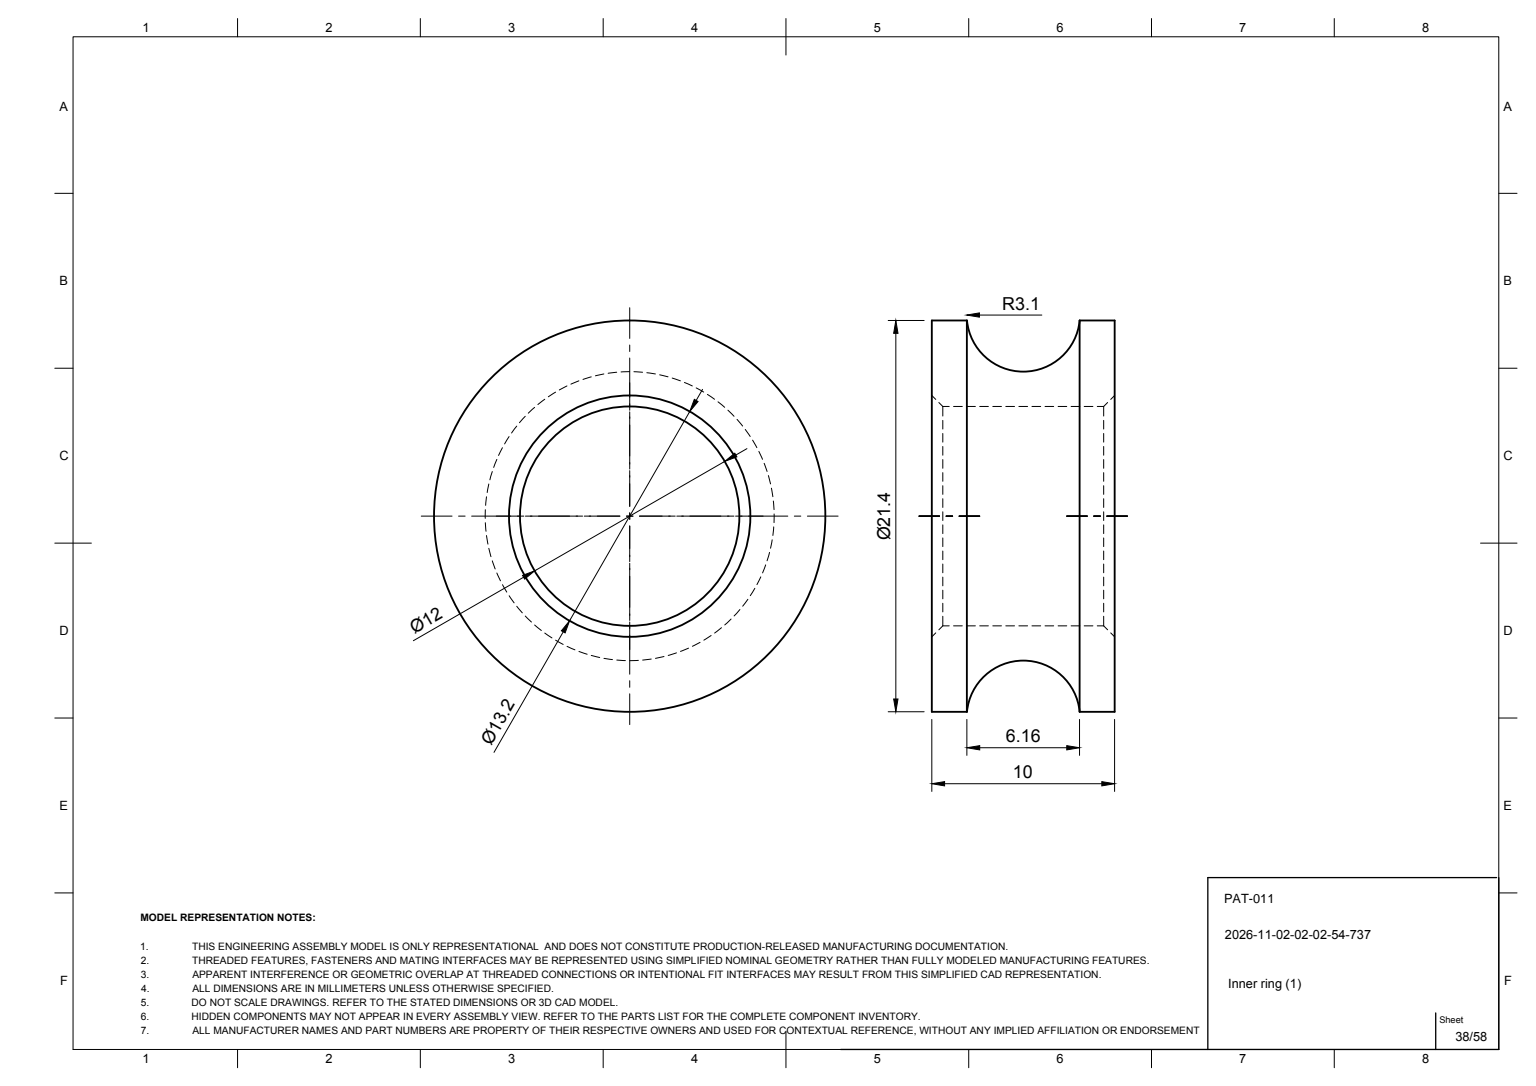
ISO-10303-21;
HEADER;
/* Generated by software containing ST-Developer
 * from STEP Tools, Inc. (www.steptools.com) 
 */

FILE_DESCRIPTION(
/* description */ ('Belt tension measurement rig'),
/* implementation_level */ '2;1');

FILE_NAME(
/* name */ 'Inner ring (1).step',
/* time_stamp */ '2026-10-28T03:24:44-07:00',
/* author */ (''),
/* organization */ (''),
/* preprocessor_version */ 'ST-DEVELOPER v20.2',
/* originating_system */ 'Autodesk Translation Framework v15.17.0.0',
/* authorisation */ '');

FILE_SCHEMA (('AUTOMOTIVE_DESIGN { 1 0 10303 214 3 1 1 }'));
ENDSEC;

DATA;
#10=MECHANICAL_DESIGN_GEOMETRIC_PRESENTATION_REPRESENTATION('',(#731),#23587);
#474=CONICAL_SURFACE('',#13666,0.63,0.785398163397448);
#475=CONICAL_SURFACE('',#13673,0.63,0.785398163397448);
#489=TOROIDAL_SURFACE('',#13655,1.1,0.309556);
#613=SHAPE_REPRESENTATION_RELATIONSHIP('SRR','None',#23862,#668);
#668=ADVANCED_BREP_SHAPE_REPRESENTATION('',(#800),#23560);
#731=STYLED_ITEM('',(#24211),#800);
#800=MANIFOLD_SOLID_BREP('Body1',#12237);
#974=FACE_BOUND('',#2589,.T.);
#975=FACE_BOUND('',#2592,.T.);
#1250=PLANE('',#13668);
#1251=PLANE('',#13671);
#1735=FACE_OUTER_BOUND('',#2584,.T.);
#1736=FACE_OUTER_BOUND('',#2585,.T.);
#1737=FACE_OUTER_BOUND('',#2586,.T.);
#1738=FACE_OUTER_BOUND('',#2587,.T.);
#1739=FACE_OUTER_BOUND('',#2588,.T.);
#1740=FACE_OUTER_BOUND('',#2590,.T.);
#1741=FACE_OUTER_BOUND('',#2591,.T.);
#1742=FACE_OUTER_BOUND('',#2593,.T.);
#2584=EDGE_LOOP('',(#9662,#9663,#9664,#9665,#9666,#9667));
#2585=EDGE_LOOP('',(#9668,#9669,#9670,#9671,#9672));
#2586=EDGE_LOOP('',(#9673,#9674,#9675,#9676));
#2587=EDGE_LOOP('',(#9677,#9678,#9679,#9680));
#2588=EDGE_LOOP('',(#9681));
#2589=EDGE_LOOP('',(#9682));
#2590=EDGE_LOOP('',(#9683,#9684,#9685,#9686,#9687));
#2591=EDGE_LOOP('',(#9688));
#2592=EDGE_LOOP('',(#9689));
#2593=EDGE_LOOP('',(#9690,#9691,#9692,#9693));
#3454=LINE('',#20863,#4205);
#3455=LINE('',#20869,#4206);
#3456=LINE('',#20873,#4207);
#3457=LINE('',#20879,#4208);
#3458=LINE('',#20884,#4209);
#4205=VECTOR('',#16575,1.070235);
#4206=VECTOR('',#16582,0.6);
#4207=VECTOR('',#16587,0.63);
#4208=VECTOR('',#16596,1.070235);
#4209=VECTOR('',#16603,0.63);
#4820=CIRCLE('',#13656,1.070235);
#4821=CIRCLE('',#13657,1.070235);
#4822=CIRCLE('',#13658,0.309556);
#4823=CIRCLE('',#13659,1.070235);
#4824=CIRCLE('',#13660,1.070235);
#4825=CIRCLE('',#13662,1.070235);
#4826=CIRCLE('',#13664,0.6);
#4827=CIRCLE('',#13665,0.6);
#4828=CIRCLE('',#13667,0.66);
#4829=CIRCLE('',#13670,1.070235);
#4830=CIRCLE('',#13672,0.66);
#5818=VERTEX_POINT('',#20852);
#5819=VERTEX_POINT('',#20853);
#5820=VERTEX_POINT('',#20856);
#5821=VERTEX_POINT('',#20858);
#5822=VERTEX_POINT('',#20862);
#5823=VERTEX_POINT('',#20866);
#5824=VERTEX_POINT('',#20868);
#5825=VERTEX_POINT('',#20872);
#5826=VERTEX_POINT('',#20877);
#5827=VERTEX_POINT('',#20881);
#7190=EDGE_CURVE('',#5818,#5819,#4820,.T.);
#7191=EDGE_CURVE('',#5819,#5818,#4821,.T.);
#7192=EDGE_CURVE('',#5819,#5820,#4822,.T.);
#7193=EDGE_CURVE('',#5821,#5820,#4823,.T.);
#7194=EDGE_CURVE('',#5820,#5821,#4824,.T.);
#7195=EDGE_CURVE('',#5821,#5822,#3454,.T.);
#7196=EDGE_CURVE('',#5822,#5822,#4825,.T.);
#7197=EDGE_CURVE('',#5823,#5823,#4826,.T.);
#7198=EDGE_CURVE('',#5823,#5824,#3455,.T.);
#7199=EDGE_CURVE('',#5824,#5824,#4827,.T.);
#7200=EDGE_CURVE('',#5824,#5825,#3456,.T.);
#7201=EDGE_CURVE('',#5825,#5825,#4828,.T.);
#7202=EDGE_CURVE('',#5826,#5826,#4829,.T.);
#7203=EDGE_CURVE('',#5826,#5818,#3457,.T.);
#7204=EDGE_CURVE('',#5827,#5827,#4830,.T.);
#7205=EDGE_CURVE('',#5827,#5823,#3458,.T.);
#9662=ORIENTED_EDGE('',*,*,#7190,.F.);
#9663=ORIENTED_EDGE('',*,*,#7191,.F.);
#9664=ORIENTED_EDGE('',*,*,#7192,.T.);
#9665=ORIENTED_EDGE('',*,*,#7193,.F.);
#9666=ORIENTED_EDGE('',*,*,#7194,.F.);
#9667=ORIENTED_EDGE('',*,*,#7192,.F.);
#9668=ORIENTED_EDGE('',*,*,#7193,.T.);
#9669=ORIENTED_EDGE('',*,*,#7194,.T.);
#9670=ORIENTED_EDGE('',*,*,#7195,.T.);
#9671=ORIENTED_EDGE('',*,*,#7196,.T.);
#9672=ORIENTED_EDGE('',*,*,#7195,.F.);
#9673=ORIENTED_EDGE('',*,*,#7197,.T.);
#9674=ORIENTED_EDGE('',*,*,#7198,.T.);
#9675=ORIENTED_EDGE('',*,*,#7199,.F.);
#9676=ORIENTED_EDGE('',*,*,#7198,.F.);
#9677=ORIENTED_EDGE('',*,*,#7199,.T.);
#9678=ORIENTED_EDGE('',*,*,#7200,.T.);
#9679=ORIENTED_EDGE('',*,*,#7201,.F.);
#9680=ORIENTED_EDGE('',*,*,#7200,.F.);
#9681=ORIENTED_EDGE('',*,*,#7196,.F.);
#9682=ORIENTED_EDGE('',*,*,#7201,.T.);
#9683=ORIENTED_EDGE('',*,*,#7202,.F.);
#9684=ORIENTED_EDGE('',*,*,#7203,.T.);
#9685=ORIENTED_EDGE('',*,*,#7190,.T.);
#9686=ORIENTED_EDGE('',*,*,#7191,.T.);
#9687=ORIENTED_EDGE('',*,*,#7203,.F.);
#9688=ORIENTED_EDGE('',*,*,#7202,.T.);
#9689=ORIENTED_EDGE('',*,*,#7204,.F.);
#9690=ORIENTED_EDGE('',*,*,#7204,.T.);
#9691=ORIENTED_EDGE('',*,*,#7205,.T.);
#9692=ORIENTED_EDGE('',*,*,#7197,.F.);
#9693=ORIENTED_EDGE('',*,*,#7205,.F.);
#11303=CYLINDRICAL_SURFACE('',#13661,1.070235);
#11304=CYLINDRICAL_SURFACE('',#13663,0.6);
#11305=CYLINDRICAL_SURFACE('',#13669,1.070235);
#11876=ADVANCED_FACE('',(#1735),#489,.F.);
#11877=ADVANCED_FACE('',(#1736),#11303,.T.);
#11878=ADVANCED_FACE('',(#1737),#11304,.F.);
#11879=ADVANCED_FACE('',(#1738),#474,.F.);
#11880=ADVANCED_FACE('',(#1739,#974),#1250,.T.);
#11881=ADVANCED_FACE('',(#1740),#11305,.T.);
#11882=ADVANCED_FACE('',(#1741,#975),#1251,.T.);
#11883=ADVANCED_FACE('',(#1742),#475,.F.);
#12237=CLOSED_SHELL('',(#11876,#11877,#11878,#11879,#11880,#11881,#11882,
#11883));
#13654=AXIS2_PLACEMENT_3D('',#20850,#16559,#16560);
#13655=AXIS2_PLACEMENT_3D('',#20851,#16561,#16562);
#13656=AXIS2_PLACEMENT_3D('',#20854,#16563,#16564);
#13657=AXIS2_PLACEMENT_3D('',#20855,#16565,#16566);
#13658=AXIS2_PLACEMENT_3D('',#20857,#16567,#16568);
#13659=AXIS2_PLACEMENT_3D('',#20859,#16569,#16570);
#13660=AXIS2_PLACEMENT_3D('',#20860,#16571,#16572);
#13661=AXIS2_PLACEMENT_3D('',#20861,#16573,#16574);
#13662=AXIS2_PLACEMENT_3D('',#20864,#16576,#16577);
#13663=AXIS2_PLACEMENT_3D('',#20865,#16578,#16579);
#13664=AXIS2_PLACEMENT_3D('',#20867,#16580,#16581);
#13665=AXIS2_PLACEMENT_3D('',#20870,#16583,#16584);
#13666=AXIS2_PLACEMENT_3D('',#20871,#16585,#16586);
#13667=AXIS2_PLACEMENT_3D('',#20874,#16588,#16589);
#13668=AXIS2_PLACEMENT_3D('',#20875,#16590,#16591);
#13669=AXIS2_PLACEMENT_3D('',#20876,#16592,#16593);
#13670=AXIS2_PLACEMENT_3D('',#20878,#16594,#16595);
#13671=AXIS2_PLACEMENT_3D('',#20880,#16597,#16598);
#13672=AXIS2_PLACEMENT_3D('',#20882,#16599,#16600);
#13673=AXIS2_PLACEMENT_3D('',#20883,#16601,#16602);
#16559=DIRECTION('axis',(0.,0.,1.));
#16560=DIRECTION('refdir',(1.,0.,0.));
#16561=DIRECTION('center_axis',(0.,-1.,0.));
#16562=DIRECTION('ref_axis',(0.,0.,-1.));
#16563=DIRECTION('center_axis',(0.,-1.,0.));
#16564=DIRECTION('ref_axis',(1.,0.,0.));
#16565=DIRECTION('center_axis',(0.,-1.,0.));
#16566=DIRECTION('ref_axis',(1.,0.,0.));
#16567=DIRECTION('center_axis',(1.,0.,1.22464679914735E-16));
#16568=DIRECTION('ref_axis',(-1.22464679914735E-16,0.,1.));
#16569=DIRECTION('center_axis',(0.,1.,0.));
#16570=DIRECTION('ref_axis',(1.,0.,0.));
#16571=DIRECTION('center_axis',(0.,1.,0.));
#16572=DIRECTION('ref_axis',(1.,0.,0.));
#16573=DIRECTION('center_axis',(0.,-1.,0.));
#16574=DIRECTION('ref_axis',(1.,0.,0.));
#16575=DIRECTION('',(0.,1.,0.));
#16576=DIRECTION('center_axis',(0.,-1.,0.));
#16577=DIRECTION('ref_axis',(1.,0.,0.));
#16578=DIRECTION('center_axis',(0.,-1.,0.));
#16579=DIRECTION('ref_axis',(1.,0.,0.));
#16580=DIRECTION('center_axis',(0.,-1.,0.));
#16581=DIRECTION('ref_axis',(1.,0.,0.));
#16582=DIRECTION('',(0.,1.,0.));
#16583=DIRECTION('center_axis',(0.,-1.,0.));
#16584=DIRECTION('ref_axis',(1.,0.,0.));
#16585=DIRECTION('center_axis',(0.,1.,0.));
#16586=DIRECTION('ref_axis',(1.,0.,0.));
#16587=DIRECTION('',(-0.707106781186548,0.707106781186547,-8.65956056235493E-17));
#16588=DIRECTION('center_axis',(0.,-1.,0.));
#16589=DIRECTION('ref_axis',(1.,0.,0.));
#16590=DIRECTION('center_axis',(0.,1.,0.));
#16591=DIRECTION('ref_axis',(0.,0.,1.));
#16592=DIRECTION('center_axis',(0.,-1.,0.));
#16593=DIRECTION('ref_axis',(1.,0.,0.));
#16594=DIRECTION('center_axis',(0.,-1.,0.));
#16595=DIRECTION('ref_axis',(1.,0.,0.));
#16596=DIRECTION('',(0.,1.,0.));
#16597=DIRECTION('center_axis',(0.,-1.,0.));
#16598=DIRECTION('ref_axis',(0.,0.,-1.));
#16599=DIRECTION('center_axis',(0.,-1.,0.));
#16600=DIRECTION('ref_axis',(1.,0.,0.));
#16601=DIRECTION('center_axis',(0.,-1.,0.));
#16602=DIRECTION('ref_axis',(1.,0.,0.));
#16603=DIRECTION('',(0.707106781186548,0.707106781186547,8.65956056235493E-17));
#20850=CARTESIAN_POINT('',(0.,0.,0.));
#20851=CARTESIAN_POINT('Origin',(0.,0.,0.));
#20852=CARTESIAN_POINT('',(-1.070235,-0.308121667383195,-1.31065986708547E-16));
#20853=CARTESIAN_POINT('',(-1.31065986708547E-16,-0.308121667383195,1.070235));
#20854=CARTESIAN_POINT('Origin',(0.,-0.308121667383195,0.));
#20855=CARTESIAN_POINT('Origin',(0.,-0.308121667383195,0.));
#20856=CARTESIAN_POINT('',(-1.31065986708547E-16,0.308121667383195,1.070235));
#20857=CARTESIAN_POINT('Origin',(-1.34711147906209E-16,0.,1.1));
#20858=CARTESIAN_POINT('',(-1.070235,0.308121667383195,1.31065986708547E-16));
#20859=CARTESIAN_POINT('Origin',(0.,0.308121667383195,0.));
#20860=CARTESIAN_POINT('Origin',(0.,0.308121667383195,0.));
#20861=CARTESIAN_POINT('Origin',(0.,0.,0.));
#20862=CARTESIAN_POINT('',(-1.070235,0.5,-1.31065986708547E-16));
#20863=CARTESIAN_POINT('',(-1.070235,0.,-1.31065986708547E-16));
#20864=CARTESIAN_POINT('Origin',(0.,0.5,0.));
#20865=CARTESIAN_POINT('Origin',(0.,0.,0.));
#20866=CARTESIAN_POINT('',(-0.6,-0.44,-7.34788079488412E-17));
#20867=CARTESIAN_POINT('Origin',(0.,-0.44,0.));
#20868=CARTESIAN_POINT('',(-0.6,0.44,-7.34788079488412E-17));
#20869=CARTESIAN_POINT('',(-0.6,0.,-7.34788079488412E-17));
#20870=CARTESIAN_POINT('Origin',(0.,0.44,0.));
#20871=CARTESIAN_POINT('Origin',(0.,0.47,0.));
#20872=CARTESIAN_POINT('',(-0.66,0.5,-8.08266887437253E-17));
#20873=CARTESIAN_POINT('',(-0.63,0.47,-7.71527483462832E-17));
#20874=CARTESIAN_POINT('Origin',(0.,0.5,0.));
#20875=CARTESIAN_POINT('Origin',(1.070235,0.5,0.));
#20876=CARTESIAN_POINT('Origin',(0.,0.,0.));
#20877=CARTESIAN_POINT('',(-1.070235,-0.5,-1.31065986708547E-16));
#20878=CARTESIAN_POINT('Origin',(0.,-0.5,0.));
#20879=CARTESIAN_POINT('',(-1.070235,0.,-1.31065986708547E-16));
#20880=CARTESIAN_POINT('Origin',(0.66,-0.5,0.));
#20881=CARTESIAN_POINT('',(-0.66,-0.5,-8.08266887437253E-17));
#20882=CARTESIAN_POINT('Origin',(0.,-0.5,0.));
#20883=CARTESIAN_POINT('Origin',(0.,-0.47,0.));
#20884=CARTESIAN_POINT('',(-0.63,-0.47,-7.71527483462832E-17));
#23495=UNCERTAINTY_MEASURE_WITH_UNIT(LENGTH_MEASURE(0.001),#23588,
'DISTANCE_ACCURACY_VALUE',
'Maximum model space distance between geometric entities at asserted c
onnectivities');
#23522=UNCERTAINTY_MEASURE_WITH_UNIT(LENGTH_MEASURE(0.001),#23588,
'DISTANCE_ACCURACY_VALUE',
'Maximum model space distance between geometric entities at asserted c
onnectivities');
#23560=(
GEOMETRIC_REPRESENTATION_CONTEXT(3)
GLOBAL_UNCERTAINTY_ASSIGNED_CONTEXT((#23495))
GLOBAL_UNIT_ASSIGNED_CONTEXT((#23588,#23590,#23591))
REPRESENTATION_CONTEXT('','3D')
);
#23587=(
GEOMETRIC_REPRESENTATION_CONTEXT(3)
GLOBAL_UNCERTAINTY_ASSIGNED_CONTEXT((#23522))
GLOBAL_UNIT_ASSIGNED_CONTEXT((#23588,#23590,#23591))
REPRESENTATION_CONTEXT('','3D')
);
#23588=(
LENGTH_UNIT()
NAMED_UNIT(*)
SI_UNIT(.CENTI.,.METRE.)
);
#23590=(
NAMED_UNIT(*)
PLANE_ANGLE_UNIT()
SI_UNIT($,.RADIAN.)
);
#23591=(
NAMED_UNIT(*)
SI_UNIT($,.STERADIAN.)
SOLID_ANGLE_UNIT()
);
#23629=SHAPE_DEFINITION_REPRESENTATION(#23701,#23862);
#23701=PRODUCT_DEFINITION_SHAPE('',$,#23927);
#23862=SHAPE_REPRESENTATION('',(#13654),#23560);
#23889=PRODUCT_DEFINITION_CONTEXT('part definition',#24083,'design');
#23927=PRODUCT_DEFINITION('Inner ring (1)','Inner ring (1)',#23991,#23889);
#23991=PRODUCT_DEFINITION_FORMATION('',$,#24122);
#24083=APPLICATION_CONTEXT(
'Core Data for Automotive Mechanical Design Process');
#24084=PRODUCT_CONTEXT('part definition',#24083,'mechanical');
#24122=PRODUCT('Inner ring (1)','Inner ring (1)','Inner ring (1)',(#24084));
#24205=COLOUR_RGB('Grey',0.48,0.52,0.57);
#24206=FILL_AREA_STYLE_COLOUR('',#24205);
#24207=FILL_AREA_STYLE('',(#24206));
#24208=SURFACE_STYLE_FILL_AREA(#24207);
#24209=SURFACE_SIDE_STYLE('',(#24208));
#24210=SURFACE_STYLE_USAGE(.BOTH.,#24209);
#24211=PRESENTATION_STYLE_ASSIGNMENT((#24210));
ENDSEC;
END-ISO-10303-21;
